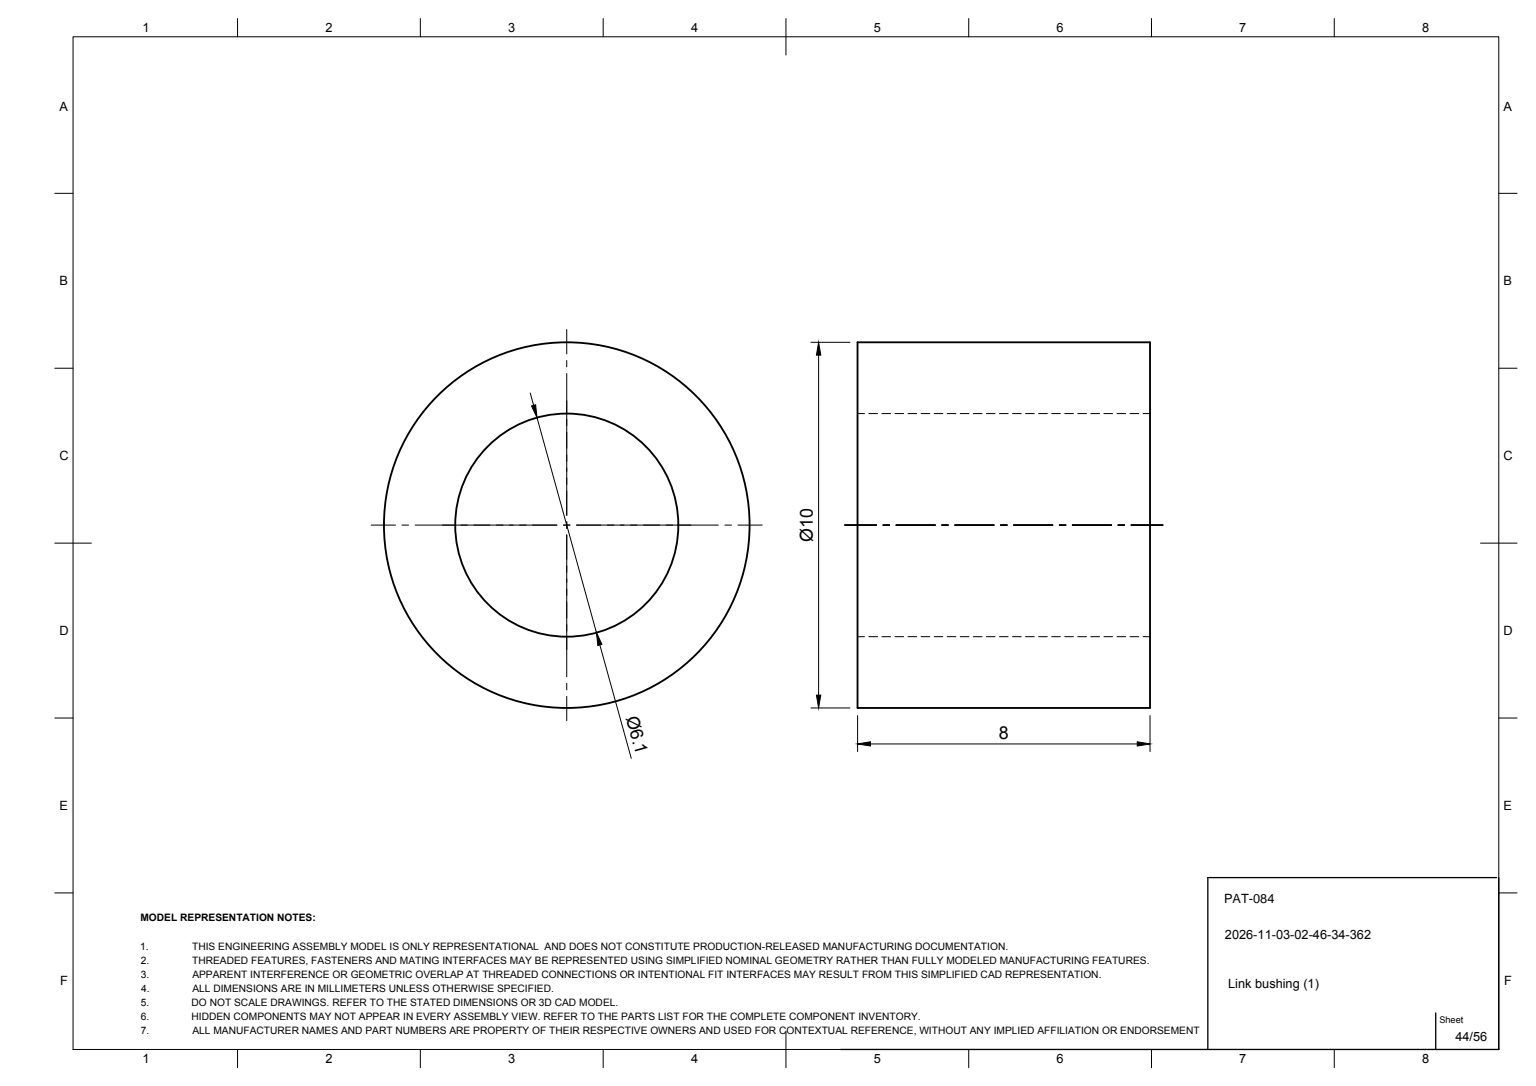
ISO-10303-21;
HEADER;
/* Generated by software containing ST-Developer
 * from STEP Tools, Inc. (www.steptools.com) 
 */

FILE_DESCRIPTION(
/* description */ ('Quick-return (Whitworth) mechanism'),
/* implementation_level */ '2;1');

FILE_NAME(
/* name */ 'Link bushing (1).step',
/* time_stamp */ '2026-10-28T03:25:57-07:00',
/* author */ (''),
/* organization */ (''),
/* preprocessor_version */ 'ST-DEVELOPER v20.2',
/* originating_system */ 'Autodesk Translation Framework v15.17.0.0',
/* authorisation */ '');

FILE_SCHEMA (('AUTOMOTIVE_DESIGN { 1 0 10303 214 3 1 1 }'));
ENDSEC;

DATA;
#10=MECHANICAL_DESIGN_GEOMETRIC_PRESENTATION_REPRESENTATION('',(#531),#14878);
#435=SHAPE_REPRESENTATION_RELATIONSHIP('SRR','None',#15108,#479);
#479=ADVANCED_BREP_SHAPE_REPRESENTATION('',(#582),#14865);
#531=STYLED_ITEM('',(#15392),#582);
#582=MANIFOLD_SOLID_BREP('Body1',#7886);
#755=FACE_BOUND('',#2036,.T.);
#756=FACE_BOUND('',#2038,.T.);
#968=PLANE('',#9144);
#969=PLANE('',#9145);
#1403=FACE_OUTER_BOUND('',#2033,.T.);
#1404=FACE_OUTER_BOUND('',#2034,.T.);
#1405=FACE_OUTER_BOUND('',#2035,.T.);
#1406=FACE_OUTER_BOUND('',#2037,.T.);
#2033=EDGE_LOOP('',(#6724,#6725,#6726,#6727));
#2034=EDGE_LOOP('',(#6728,#6729,#6730,#6731));
#2035=EDGE_LOOP('',(#6732));
#2036=EDGE_LOOP('',(#6733));
#2037=EDGE_LOOP('',(#6734));
#2038=EDGE_LOOP('',(#6735));
#2514=LINE('',#14177,#3037);
#2515=LINE('',#14183,#3038);
#3037=VECTOR('',#11253,0.305);
#3038=VECTOR('',#11260,0.5);
#3567=CIRCLE('',#9139,0.305);
#3568=CIRCLE('',#9140,0.305);
#3569=CIRCLE('',#9142,0.5);
#3570=CIRCLE('',#9143,0.5);
#4128=VERTEX_POINT('',#14174);
#4129=VERTEX_POINT('',#14176);
#4130=VERTEX_POINT('',#14180);
#4131=VERTEX_POINT('',#14182);
#5019=EDGE_CURVE('',#4128,#4128,#3567,.T.);
#5020=EDGE_CURVE('',#4128,#4129,#2514,.T.);
#5021=EDGE_CURVE('',#4129,#4129,#3568,.T.);
#5022=EDGE_CURVE('',#4130,#4130,#3569,.T.);
#5023=EDGE_CURVE('',#4130,#4131,#2515,.T.);
#5024=EDGE_CURVE('',#4131,#4131,#3570,.T.);
#6724=ORIENTED_EDGE('',*,*,#5019,.F.);
#6725=ORIENTED_EDGE('',*,*,#5020,.T.);
#6726=ORIENTED_EDGE('',*,*,#5021,.T.);
#6727=ORIENTED_EDGE('',*,*,#5020,.F.);
#6728=ORIENTED_EDGE('',*,*,#5022,.F.);
#6729=ORIENTED_EDGE('',*,*,#5023,.T.);
#6730=ORIENTED_EDGE('',*,*,#5024,.T.);
#6731=ORIENTED_EDGE('',*,*,#5023,.F.);
#6732=ORIENTED_EDGE('',*,*,#5022,.T.);
#6733=ORIENTED_EDGE('',*,*,#5019,.T.);
#6734=ORIENTED_EDGE('',*,*,#5024,.F.);
#6735=ORIENTED_EDGE('',*,*,#5021,.F.);
#7353=CYLINDRICAL_SURFACE('',#9138,0.305);
#7354=CYLINDRICAL_SURFACE('',#9141,0.5);
#7734=ADVANCED_FACE('',(#1403),#7353,.F.);
#7735=ADVANCED_FACE('',(#1404),#7354,.T.);
#7736=ADVANCED_FACE('',(#1405,#755),#968,.T.);
#7737=ADVANCED_FACE('',(#1406,#756),#969,.F.);
#7886=CLOSED_SHELL('',(#7734,#7735,#7736,#7737));
#9137=AXIS2_PLACEMENT_3D('',#14172,#11247,#11248);
#9138=AXIS2_PLACEMENT_3D('',#14173,#11249,#11250);
#9139=AXIS2_PLACEMENT_3D('',#14175,#11251,#11252);
#9140=AXIS2_PLACEMENT_3D('',#14178,#11254,#11255);
#9141=AXIS2_PLACEMENT_3D('',#14179,#11256,#11257);
#9142=AXIS2_PLACEMENT_3D('',#14181,#11258,#11259);
#9143=AXIS2_PLACEMENT_3D('',#14184,#11261,#11262);
#9144=AXIS2_PLACEMENT_3D('',#14185,#11263,#11264);
#9145=AXIS2_PLACEMENT_3D('',#14186,#11265,#11266);
#11247=DIRECTION('axis',(0.,0.,1.));
#11248=DIRECTION('refdir',(1.,0.,0.));
#11249=DIRECTION('center_axis',(0.,0.,1.));
#11250=DIRECTION('ref_axis',(1.,0.,0.));
#11251=DIRECTION('center_axis',(0.,0.,-1.));
#11252=DIRECTION('ref_axis',(1.,0.,0.));
#11253=DIRECTION('',(0.,0.,-1.));
#11254=DIRECTION('center_axis',(0.,0.,-1.));
#11255=DIRECTION('ref_axis',(1.,0.,0.));
#11256=DIRECTION('center_axis',(0.,0.,1.));
#11257=DIRECTION('ref_axis',(1.,0.,0.));
#11258=DIRECTION('center_axis',(0.,0.,1.));
#11259=DIRECTION('ref_axis',(1.,0.,0.));
#11260=DIRECTION('',(0.,0.,-1.));
#11261=DIRECTION('center_axis',(0.,0.,1.));
#11262=DIRECTION('ref_axis',(1.,0.,0.));
#11263=DIRECTION('center_axis',(0.,0.,1.));
#11264=DIRECTION('ref_axis',(1.,0.,0.));
#11265=DIRECTION('center_axis',(0.,0.,1.));
#11266=DIRECTION('ref_axis',(1.,0.,0.));
#14172=CARTESIAN_POINT('',(0.,0.,0.));
#14173=CARTESIAN_POINT('Origin',(9.16515138991168,16.,8.4));
#14174=CARTESIAN_POINT('',(8.86015138991168,16.,9.2));
#14175=CARTESIAN_POINT('Origin',(9.16515138991168,16.,9.2));
#14176=CARTESIAN_POINT('',(8.86015138991168,16.,8.4));
#14177=CARTESIAN_POINT('',(8.86015138991168,16.,8.4));
#14178=CARTESIAN_POINT('Origin',(9.16515138991168,16.,8.4));
#14179=CARTESIAN_POINT('Origin',(9.16515138991168,16.,8.4));
#14180=CARTESIAN_POINT('',(8.66515138991168,16.,9.2));
#14181=CARTESIAN_POINT('Origin',(9.16515138991168,16.,9.2));
#14182=CARTESIAN_POINT('',(8.66515138991168,16.,8.4));
#14183=CARTESIAN_POINT('',(8.66515138991168,16.,8.4));
#14184=CARTESIAN_POINT('Origin',(9.16515138991168,16.,8.4));
#14185=CARTESIAN_POINT('Origin',(9.16515138991168,16.,9.2));
#14186=CARTESIAN_POINT('Origin',(9.16515138991168,16.,8.4));
#14811=UNCERTAINTY_MEASURE_WITH_UNIT(LENGTH_MEASURE(0.001),#14879,
'DISTANCE_ACCURACY_VALUE',
'Maximum model space distance between geometric entities at asserted c
onnectivities');
#14824=UNCERTAINTY_MEASURE_WITH_UNIT(LENGTH_MEASURE(0.001),#14879,
'DISTANCE_ACCURACY_VALUE',
'Maximum model space distance between geometric entities at asserted c
onnectivities');
#14865=(
GEOMETRIC_REPRESENTATION_CONTEXT(3)
GLOBAL_UNCERTAINTY_ASSIGNED_CONTEXT((#14811))
GLOBAL_UNIT_ASSIGNED_CONTEXT((#14879,#14881,#14882))
REPRESENTATION_CONTEXT('','3D')
);
#14878=(
GEOMETRIC_REPRESENTATION_CONTEXT(3)
GLOBAL_UNCERTAINTY_ASSIGNED_CONTEXT((#14824))
GLOBAL_UNIT_ASSIGNED_CONTEXT((#14879,#14881,#14882))
REPRESENTATION_CONTEXT('','3D')
);
#14879=(
LENGTH_UNIT()
NAMED_UNIT(*)
SI_UNIT(.CENTI.,.METRE.)
);
#14881=(
NAMED_UNIT(*)
PLANE_ANGLE_UNIT()
SI_UNIT($,.RADIAN.)
);
#14882=(
NAMED_UNIT(*)
SI_UNIT($,.STERADIAN.)
SOLID_ANGLE_UNIT()
);
#14923=SHAPE_DEFINITION_REPRESENTATION(#14982,#15108);
#14982=PRODUCT_DEFINITION_SHAPE('',$,#15162);
#15108=SHAPE_REPRESENTATION('',(#9137),#14865);
#15121=PRODUCT_DEFINITION_CONTEXT('part definition',#15282,'design');
#15162=PRODUCT_DEFINITION('Link bushing (1)','Link bushing (1)',#15215,#15121);
#15215=PRODUCT_DEFINITION_FORMATION('',$,#15324);
#15282=APPLICATION_CONTEXT(
'Core Data for Automotive Mechanical Design Process');
#15283=PRODUCT_CONTEXT('part definition',#15282,'mechanical');
#15324=PRODUCT('Link bushing (1)','Link bushing (1)','Link bushing (1)',(#15283));
#15386=COLOUR_RGB('Light Blue',0.38,0.62,0.78);
#15387=FILL_AREA_STYLE_COLOUR('',#15386);
#15388=FILL_AREA_STYLE('',(#15387));
#15389=SURFACE_STYLE_FILL_AREA(#15388);
#15390=SURFACE_SIDE_STYLE('',(#15389));
#15391=SURFACE_STYLE_USAGE(.BOTH.,#15390);
#15392=PRESENTATION_STYLE_ASSIGNMENT((#15391));
ENDSEC;
END-ISO-10303-21;
